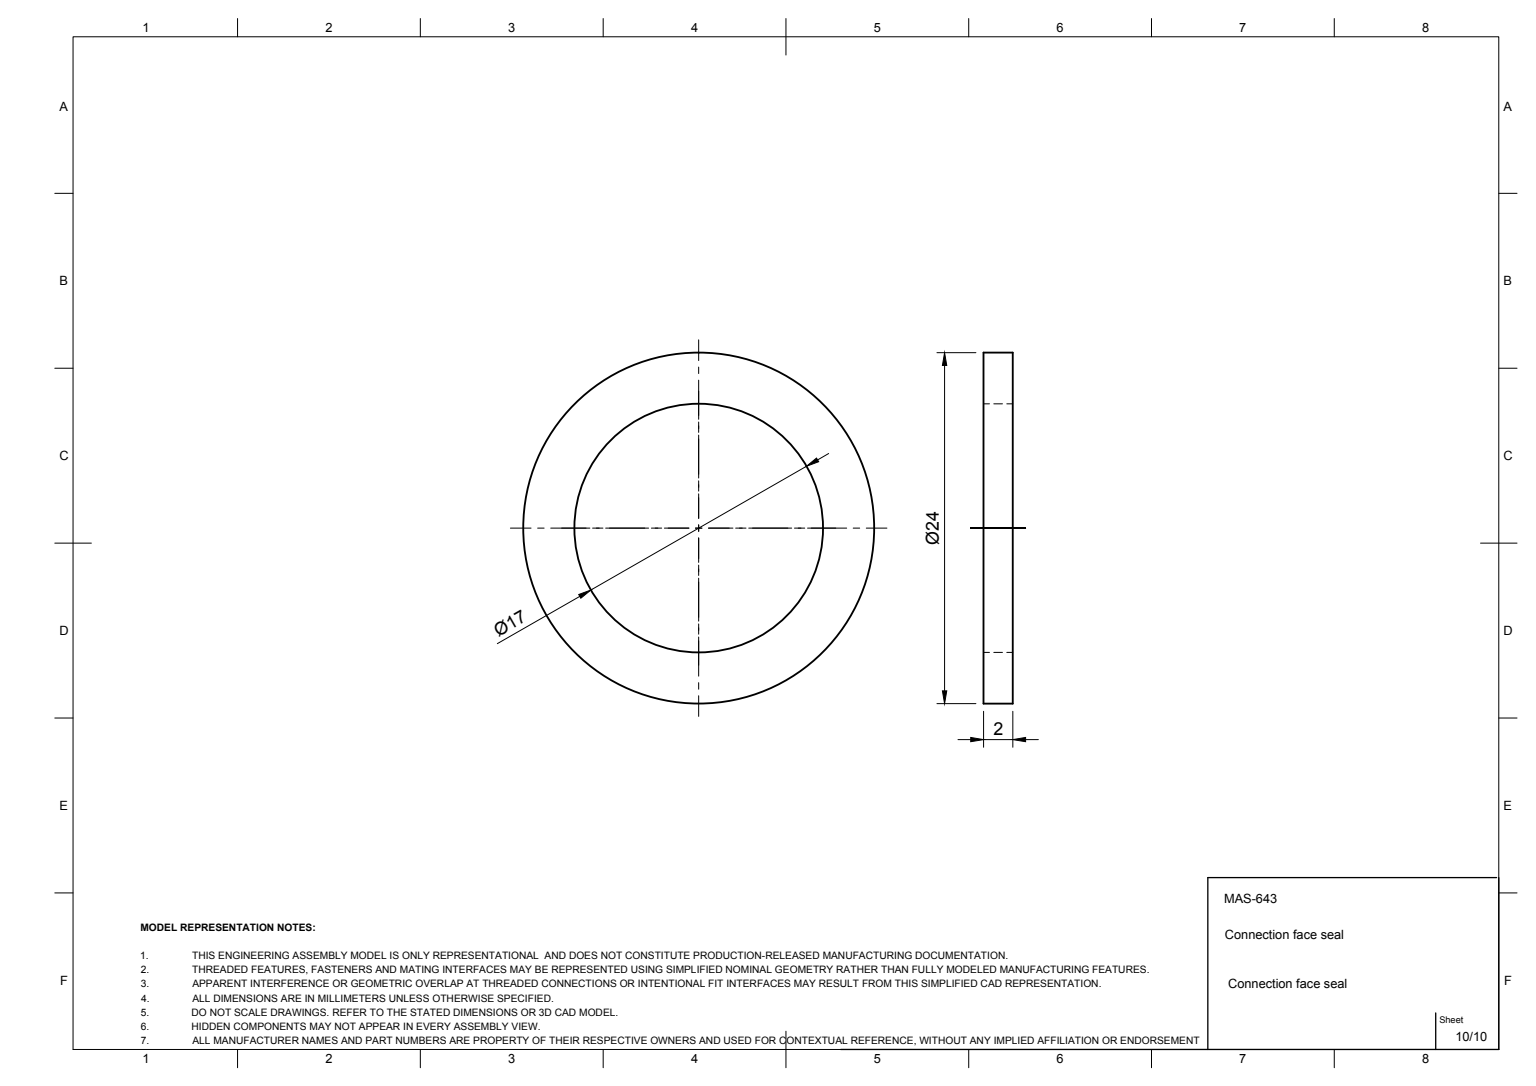
ISO-10303-21;
HEADER;
/* Generated by software containing ST-Developer
 * from STEP Tools, Inc. (www.steptools.com) 
 */

FILE_DESCRIPTION(
/* description */ ('Independent eighteen-tube parallel-flow evaporator geometry. Repeated
 machined headers and gasketed service covers, eighteen copper tubes, 
twenty-nine punched fins, threaded hose connections and bolted mountin
g feet. Native editable features and instanced parts. Braze details, w
orking fluid, pressure and thermal ratings require engineering selecti
on.'),
/* implementation_level */ '2;1');

FILE_NAME(
/* name */ 'Connection face seal.step',
/* time_stamp */ '2026-11-08T20:53:59-08:00',
/* author */ (''),
/* organization */ (''),
/* preprocessor_version */ 'ST-DEVELOPER v20.2',
/* originating_system */ 'Autodesk Translation Framework v15.17.0.0',
/* authorisation */ '');

FILE_SCHEMA (('AUTOMOTIVE_DESIGN { 1 0 10303 214 3 1 1 }'));
ENDSEC;

DATA;
#10=MECHANICAL_DESIGN_GEOMETRIC_PRESENTATION_REPRESENTATION('',(#342),#42620);
#322=SHAPE_REPRESENTATION_RELATIONSHIP('SRR','None',#42732,#332);
#332=ADVANCED_BREP_SHAPE_REPRESENTATION('',(#352),#42619);
#342=STYLED_ITEM('',(#42788),#352);
#352=MANIFOLD_SOLID_BREP('Body1',#10392);
#485=FACE_BOUND('',#1822,.T.);
#486=FACE_BOUND('',#1824,.T.);
#577=PLANE('',#11229);
#578=PLANE('',#11230);
#1143=FACE_OUTER_BOUND('',#1819,.T.);
#1144=FACE_OUTER_BOUND('',#1820,.T.);
#1145=FACE_OUTER_BOUND('',#1821,.T.);
#1146=FACE_OUTER_BOUND('',#1823,.T.);
#1819=EDGE_LOOP('',(#9401,#9402,#9403,#9404));
#1820=EDGE_LOOP('',(#9405,#9406,#9407,#9408));
#1821=EDGE_LOOP('',(#9409));
#1822=EDGE_LOOP('',(#9410));
#1823=EDGE_LOOP('',(#9411));
#1824=EDGE_LOOP('',(#9412));
#2017=CIRCLE('',#11224,8.5);
#2018=CIRCLE('',#11225,8.5);
#2019=CIRCLE('',#11227,12.);
#2020=CIRCLE('',#11228,12.);
#3335=LINE('',#42512,#3873);
#3336=LINE('',#42518,#3874);
#3873=VECTOR('',#13284,8.5);
#3874=VECTOR('',#13291,12.);
#4873=VERTEX_POINT('',#42509);
#4874=VERTEX_POINT('',#42511);
#4875=VERTEX_POINT('',#42515);
#4876=VERTEX_POINT('',#42517);
#6383=EDGE_CURVE('',#4873,#4873,#2017,.T.);
#6384=EDGE_CURVE('',#4873,#4874,#3335,.T.);
#6385=EDGE_CURVE('',#4874,#4874,#2018,.T.);
#6386=EDGE_CURVE('',#4875,#4875,#2019,.T.);
#6387=EDGE_CURVE('',#4875,#4876,#3336,.T.);
#6388=EDGE_CURVE('',#4876,#4876,#2020,.T.);
#9401=ORIENTED_EDGE('',*,*,#6383,.F.);
#9402=ORIENTED_EDGE('',*,*,#6384,.T.);
#9403=ORIENTED_EDGE('',*,*,#6385,.T.);
#9404=ORIENTED_EDGE('',*,*,#6384,.F.);
#9405=ORIENTED_EDGE('',*,*,#6386,.F.);
#9406=ORIENTED_EDGE('',*,*,#6387,.T.);
#9407=ORIENTED_EDGE('',*,*,#6388,.T.);
#9408=ORIENTED_EDGE('',*,*,#6387,.F.);
#9409=ORIENTED_EDGE('',*,*,#6386,.T.);
#9410=ORIENTED_EDGE('',*,*,#6383,.T.);
#9411=ORIENTED_EDGE('',*,*,#6388,.F.);
#9412=ORIENTED_EDGE('',*,*,#6385,.F.);
#9837=CYLINDRICAL_SURFACE('',#11223,8.5);
#9838=CYLINDRICAL_SURFACE('',#11226,12.);
#10379=ADVANCED_FACE('',(#1143),#9837,.F.);
#10380=ADVANCED_FACE('',(#1144),#9838,.T.);
#10381=ADVANCED_FACE('',(#1145,#485),#577,.T.);
#10382=ADVANCED_FACE('',(#1146,#486),#578,.F.);
#10392=CLOSED_SHELL('',(#10379,#10380,#10381,#10382));
#11222=AXIS2_PLACEMENT_3D('',#42507,#13278,#13279);
#11223=AXIS2_PLACEMENT_3D('',#42508,#13280,#13281);
#11224=AXIS2_PLACEMENT_3D('',#42510,#13282,#13283);
#11225=AXIS2_PLACEMENT_3D('',#42513,#13285,#13286);
#11226=AXIS2_PLACEMENT_3D('',#42514,#13287,#13288);
#11227=AXIS2_PLACEMENT_3D('',#42516,#13289,#13290);
#11228=AXIS2_PLACEMENT_3D('',#42519,#13292,#13293);
#11229=AXIS2_PLACEMENT_3D('',#42520,#13294,#13295);
#11230=AXIS2_PLACEMENT_3D('',#42521,#13296,#13297);
#13278=DIRECTION('axis',(0.,0.,1.));
#13279=DIRECTION('refdir',(1.,0.,0.));
#13280=DIRECTION('center_axis',(0.,0.,1.));
#13281=DIRECTION('ref_axis',(1.,0.,0.));
#13282=DIRECTION('center_axis',(0.,0.,-1.));
#13283=DIRECTION('ref_axis',(1.,0.,0.));
#13284=DIRECTION('',(0.,0.,-1.));
#13285=DIRECTION('center_axis',(0.,0.,-1.));
#13286=DIRECTION('ref_axis',(1.,0.,0.));
#13287=DIRECTION('center_axis',(0.,0.,1.));
#13288=DIRECTION('ref_axis',(1.,0.,0.));
#13289=DIRECTION('center_axis',(0.,0.,1.));
#13290=DIRECTION('ref_axis',(1.,0.,0.));
#13291=DIRECTION('',(0.,0.,-1.));
#13292=DIRECTION('center_axis',(0.,0.,1.));
#13293=DIRECTION('ref_axis',(1.,0.,0.));
#13294=DIRECTION('center_axis',(0.,0.,1.));
#13295=DIRECTION('ref_axis',(1.,0.,0.));
#13296=DIRECTION('center_axis',(0.,0.,1.));
#13297=DIRECTION('ref_axis',(1.,0.,0.));
#42507=CARTESIAN_POINT('',(0.,0.,0.));
#42508=CARTESIAN_POINT('Origin',(0.,0.,-50.));
#42509=CARTESIAN_POINT('',(-8.5,-1.04094977927525E-15,-48.));
#42510=CARTESIAN_POINT('Origin',(0.,0.,-48.));
#42511=CARTESIAN_POINT('',(-8.5,-1.04094977927525E-15,-50.));
#42512=CARTESIAN_POINT('',(-8.5,-1.04094977927525E-15,-50.));
#42513=CARTESIAN_POINT('Origin',(0.,0.,-50.));
#42514=CARTESIAN_POINT('Origin',(0.,0.,-50.));
#42515=CARTESIAN_POINT('',(-12.,-1.46957615897682E-15,-48.));
#42516=CARTESIAN_POINT('Origin',(0.,0.,-48.));
#42517=CARTESIAN_POINT('',(-12.,-1.46957615897682E-15,-50.));
#42518=CARTESIAN_POINT('',(-12.,-1.46957615897682E-15,-50.));
#42519=CARTESIAN_POINT('Origin',(0.,0.,-50.));
#42520=CARTESIAN_POINT('Origin',(0.,0.,-48.));
#42521=CARTESIAN_POINT('Origin',(0.,0.,-50.));
#42607=UNCERTAINTY_MEASURE_WITH_UNIT(LENGTH_MEASURE(0.01),#42621,
'DISTANCE_ACCURACY_VALUE',
'Maximum model space distance between geometric entities at asserted c
onnectivities');
#42608=UNCERTAINTY_MEASURE_WITH_UNIT(LENGTH_MEASURE(0.01),#42621,
'DISTANCE_ACCURACY_VALUE',
'Maximum model space distance between geometric entities at asserted c
onnectivities');
#42619=(
GEOMETRIC_REPRESENTATION_CONTEXT(3)
GLOBAL_UNCERTAINTY_ASSIGNED_CONTEXT((#42607))
GLOBAL_UNIT_ASSIGNED_CONTEXT((#42621,#42623,#42624))
REPRESENTATION_CONTEXT('','3D')
);
#42620=(
GEOMETRIC_REPRESENTATION_CONTEXT(3)
GLOBAL_UNCERTAINTY_ASSIGNED_CONTEXT((#42608))
GLOBAL_UNIT_ASSIGNED_CONTEXT((#42621,#42623,#42624))
REPRESENTATION_CONTEXT('','3D')
);
#42621=(
LENGTH_UNIT()
NAMED_UNIT(*)
SI_UNIT(.MILLI.,.METRE.)
);
#42623=(
NAMED_UNIT(*)
PLANE_ANGLE_UNIT()
SI_UNIT($,.RADIAN.)
);
#42624=(
NAMED_UNIT(*)
SI_UNIT($,.STERADIAN.)
SOLID_ANGLE_UNIT()
);
#42635=SHAPE_DEFINITION_REPRESENTATION(#42646,#42732);
#42646=PRODUCT_DEFINITION_SHAPE('',$,#42744);
#42732=SHAPE_REPRESENTATION('',(#11222),#42619);
#42733=PRODUCT_DEFINITION_CONTEXT('part definition',#42768,'design');
#42744=PRODUCT_DEFINITION('Connection face seal','Connection face seal',
#42755,#42733);
#42755=PRODUCT_DEFINITION_FORMATION('',$,#42780);
#42768=APPLICATION_CONTEXT(
'Core Data for Automotive Mechanical Design Process');
#42769=PRODUCT_CONTEXT('part definition',#42768,'mechanical');
#42780=PRODUCT('Connection face seal','Connection face seal',$,(#42769));
#42788=PRESENTATION_STYLE_ASSIGNMENT((#42796));
#42796=SURFACE_STYLE_USAGE(.BOTH.,#42804);
#42804=SURFACE_SIDE_STYLE('',(#42812));
#42812=SURFACE_STYLE_FILL_AREA(#42820);
#42820=FILL_AREA_STYLE('Black',(#42828));
#42828=FILL_AREA_STYLE_COLOUR('Black',#42836);
#42836=COLOUR_RGB('Black',0.137254901960784,0.152941176470588,0.176470588235294);
ENDSEC;
END-ISO-10303-21;
